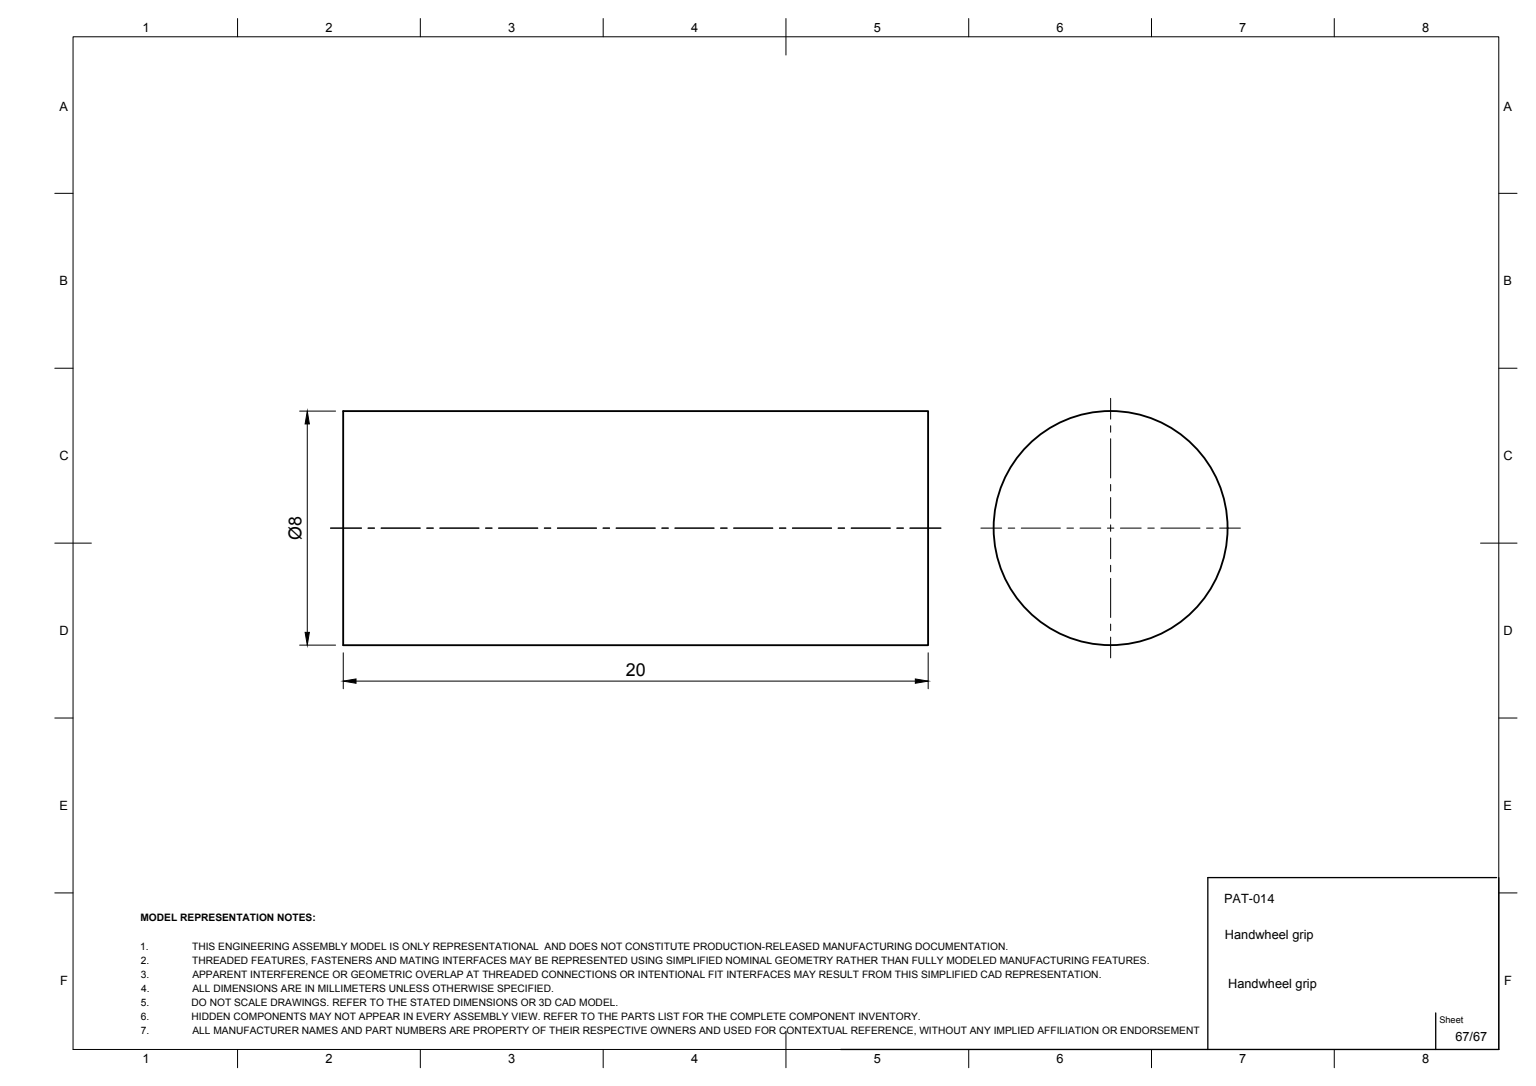
ISO-10303-21;
HEADER;
/* Generated by software containing ST-Developer
 * from STEP Tools, Inc. (www.steptools.com) 
 */

FILE_DESCRIPTION(
/* description */ ('Bin tilter linkage'),
/* implementation_level */ '2;1');

FILE_NAME(
/* name */ 'Handwheel grip.step',
/* time_stamp */ '2026-10-28T03:26:24-07:00',
/* author */ (''),
/* organization */ (''),
/* preprocessor_version */ 'ST-DEVELOPER v20.2',
/* originating_system */ 'Autodesk Translation Framework v15.17.0.0',
/* authorisation */ '');

FILE_SCHEMA (('AUTOMOTIVE_DESIGN { 1 0 10303 214 3 1 1 }'));
ENDSEC;

DATA;
#10=MECHANICAL_DESIGN_GEOMETRIC_PRESENTATION_REPRESENTATION('',(#975),#23728);
#755=SHAPE_REPRESENTATION_RELATIONSHIP('SRR','None',#24227,#861);
#861=ADVANCED_BREP_SHAPE_REPRESENTATION('',(#1086),#23727);
#975=STYLED_ITEM('',(#24772),#1086);
#1086=MANIFOLD_SOLID_BREP('Body1',#12508);
#1888=PLANE('',#15460);
#1889=PLANE('',#15461);
#2664=FACE_OUTER_BOUND('',#3846,.T.);
#2665=FACE_OUTER_BOUND('',#3847,.T.);
#2666=FACE_OUTER_BOUND('',#3848,.T.);
#3846=EDGE_LOOP('',(#11261,#11262,#11263,#11264));
#3847=EDGE_LOOP('',(#11265));
#3848=EDGE_LOOP('',(#11266));
#4523=LINE('',#23479,#5198);
#5198=VECTOR('',#19714,0.4);
#5955=CIRCLE('',#15458,0.4);
#5956=CIRCLE('',#15459,0.4);
#6924=VERTEX_POINT('',#23476);
#6925=VERTEX_POINT('',#23478);
#8370=EDGE_CURVE('',#6924,#6924,#5955,.T.);
#8371=EDGE_CURVE('',#6924,#6925,#4523,.T.);
#8372=EDGE_CURVE('',#6925,#6925,#5956,.T.);
#11261=ORIENTED_EDGE('',*,*,#8370,.F.);
#11262=ORIENTED_EDGE('',*,*,#8371,.T.);
#11263=ORIENTED_EDGE('',*,*,#8372,.T.);
#11264=ORIENTED_EDGE('',*,*,#8371,.F.);
#11265=ORIENTED_EDGE('',*,*,#8370,.T.);
#11266=ORIENTED_EDGE('',*,*,#8372,.F.);
#11614=CYLINDRICAL_SURFACE('',#15457,0.4);
#12389=ADVANCED_FACE('',(#2664),#11614,.T.);
#12390=ADVANCED_FACE('',(#2665),#1888,.T.);
#12391=ADVANCED_FACE('',(#2666),#1889,.F.);
#12508=CLOSED_SHELL('',(#12389,#12390,#12391));
#15456=AXIS2_PLACEMENT_3D('',#23474,#19708,#19709);
#15457=AXIS2_PLACEMENT_3D('',#23475,#19710,#19711);
#15458=AXIS2_PLACEMENT_3D('',#23477,#19712,#19713);
#15459=AXIS2_PLACEMENT_3D('',#23480,#19715,#19716);
#15460=AXIS2_PLACEMENT_3D('',#23481,#19717,#19718);
#15461=AXIS2_PLACEMENT_3D('',#23482,#19719,#19720);
#19708=DIRECTION('axis',(0.,0.,1.));
#19709=DIRECTION('refdir',(1.,0.,0.));
#19710=DIRECTION('center_axis',(1.,0.,0.));
#19711=DIRECTION('ref_axis',(0.,0.,-1.));
#19712=DIRECTION('center_axis',(1.,0.,0.));
#19713=DIRECTION('ref_axis',(0.,0.,-1.));
#19714=DIRECTION('',(-1.,0.,0.));
#19715=DIRECTION('center_axis',(1.,0.,0.));
#19716=DIRECTION('ref_axis',(0.,0.,-1.));
#19717=DIRECTION('center_axis',(1.,0.,0.));
#19718=DIRECTION('ref_axis',(0.,0.,-1.));
#19719=DIRECTION('center_axis',(1.,0.,0.));
#19720=DIRECTION('ref_axis',(0.,0.,-1.));
#23474=CARTESIAN_POINT('',(0.,0.,0.));
#23475=CARTESIAN_POINT('Origin',(-14.5,-4.5,9.5));
#23476=CARTESIAN_POINT('',(-12.5,-4.5,9.9));
#23477=CARTESIAN_POINT('Origin',(-12.5,-4.5,9.5));
#23478=CARTESIAN_POINT('',(-14.5,-4.5,9.9));
#23479=CARTESIAN_POINT('',(-14.5,-4.5,9.9));
#23480=CARTESIAN_POINT('Origin',(-14.5,-4.5,9.5));
#23481=CARTESIAN_POINT('Origin',(-12.5,-4.5,9.5));
#23482=CARTESIAN_POINT('Origin',(-14.5,-4.5,9.5));
#23610=UNCERTAINTY_MEASURE_WITH_UNIT(LENGTH_MEASURE(0.001),#23729,
'DISTANCE_ACCURACY_VALUE',
'Maximum model space distance between geometric entities at asserted c
onnectivities');
#23611=UNCERTAINTY_MEASURE_WITH_UNIT(LENGTH_MEASURE(0.001),#23729,
'DISTANCE_ACCURACY_VALUE',
'Maximum model space distance between geometric entities at asserted c
onnectivities');
#23727=(
GEOMETRIC_REPRESENTATION_CONTEXT(3)
GLOBAL_UNCERTAINTY_ASSIGNED_CONTEXT((#23610))
GLOBAL_UNIT_ASSIGNED_CONTEXT((#23729,#23731,#23732))
REPRESENTATION_CONTEXT('','3D')
);
#23728=(
GEOMETRIC_REPRESENTATION_CONTEXT(3)
GLOBAL_UNCERTAINTY_ASSIGNED_CONTEXT((#23611))
GLOBAL_UNIT_ASSIGNED_CONTEXT((#23729,#23731,#23732))
REPRESENTATION_CONTEXT('','3D')
);
#23729=(
LENGTH_UNIT()
NAMED_UNIT(*)
SI_UNIT(.CENTI.,.METRE.)
);
#23731=(
NAMED_UNIT(*)
PLANE_ANGLE_UNIT()
SI_UNIT($,.RADIAN.)
);
#23732=(
NAMED_UNIT(*)
SI_UNIT($,.STERADIAN.)
SOLID_ANGLE_UNIT()
);
#23848=SHAPE_DEFINITION_REPRESENTATION(#24099,#24227);
#24099=PRODUCT_DEFINITION_SHAPE('',$,#24344);
#24227=SHAPE_REPRESENTATION('',(#15456),#23727);
#24228=PRODUCT_DEFINITION_CONTEXT('part definition',#24578,'design');
#24344=PRODUCT_DEFINITION('Handwheel grip','Handwheel grip',#24460,#24228);
#24460=PRODUCT_DEFINITION_FORMATION('',$,#24695);
#24578=APPLICATION_CONTEXT(
'Core Data for Automotive Mechanical Design Process');
#24579=PRODUCT_CONTEXT('part definition',#24578,'mechanical');
#24695=PRODUCT('Handwheel grip','Handwheel grip','Handwheel grip',(#24579));
#24766=COLOUR_RGB('Black',0.12,0.14,0.17);
#24767=FILL_AREA_STYLE_COLOUR('',#24766);
#24768=FILL_AREA_STYLE('',(#24767));
#24769=SURFACE_STYLE_FILL_AREA(#24768);
#24770=SURFACE_SIDE_STYLE('',(#24769));
#24771=SURFACE_STYLE_USAGE(.BOTH.,#24770);
#24772=PRESENTATION_STYLE_ASSIGNMENT((#24771));
ENDSEC;
END-ISO-10303-21;
